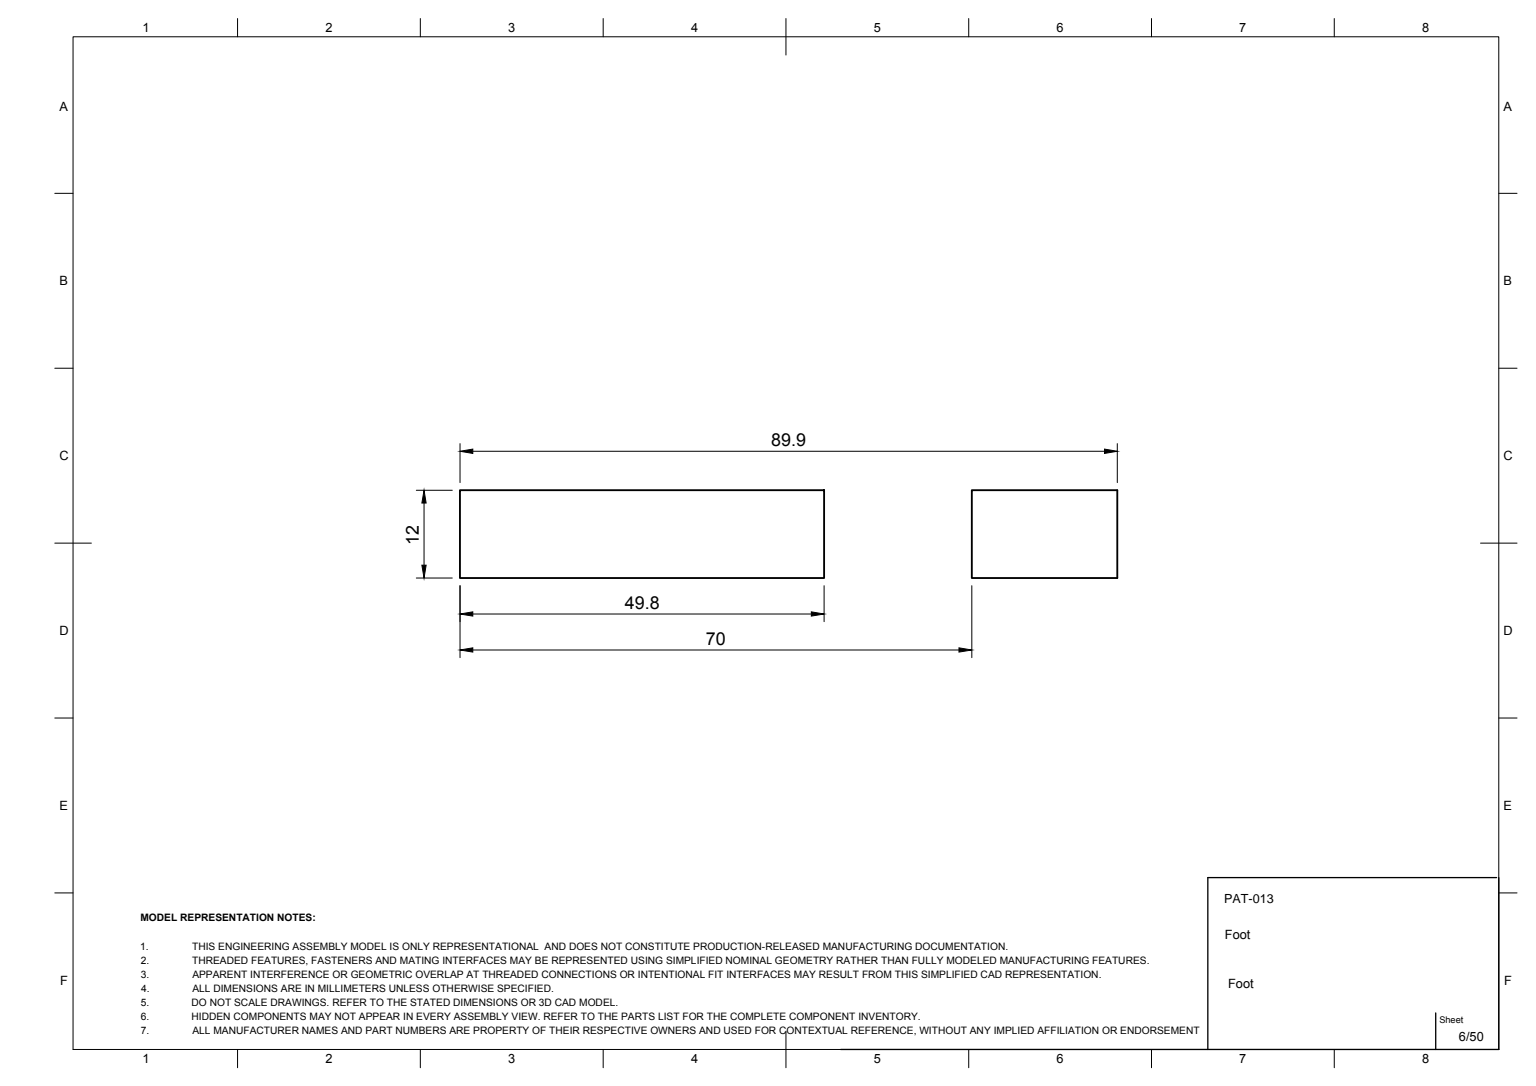
ISO-10303-21;
HEADER;
/* Generated by software containing ST-Developer
 * from STEP Tools, Inc. (www.steptools.com) 
 */

FILE_DESCRIPTION(
/* description */ ('Belt-driven linear axis on 2020 extrusion'),
/* implementation_level */ '2;1');

FILE_NAME(
/* name */ 'Foot.step',
/* time_stamp */ '2026-10-28T03:26:09-07:00',
/* author */ (''),
/* organization */ (''),
/* preprocessor_version */ 'ST-DEVELOPER v20.2',
/* originating_system */ 'Autodesk Translation Framework v15.17.0.0',
/* authorisation */ '');

FILE_SCHEMA (('AUTOMOTIVE_DESIGN { 1 0 10303 214 3 1 1 }'));
ENDSEC;

DATA;
#10=MECHANICAL_DESIGN_GEOMETRIC_PRESENTATION_REPRESENTATION('',(#611,#612),#20096);
#519=SHAPE_REPRESENTATION_RELATIONSHIP('SRR','None',#20315,#565);
#565=ADVANCED_BREP_SHAPE_REPRESENTATION('',(#667,#668),#20046);
#611=STYLED_ITEM('',(#20664),#667);
#612=STYLED_ITEM('',(#20664),#668);
#667=MANIFOLD_SOLID_BREP('Body1',#10924);
#668=MANIFOLD_SOLID_BREP('Body2',#10925);
#911=PLANE('',#11576);
#912=PLANE('',#11577);
#913=PLANE('',#11578);
#914=PLANE('',#11579);
#915=PLANE('',#11580);
#916=PLANE('',#11581);
#917=PLANE('',#11582);
#918=PLANE('',#11583);
#919=PLANE('',#11584);
#920=PLANE('',#11585);
#921=PLANE('',#11586);
#922=PLANE('',#11587);
#1292=FACE_OUTER_BOUND('',#1938,.T.);
#1293=FACE_OUTER_BOUND('',#1939,.T.);
#1294=FACE_OUTER_BOUND('',#1940,.T.);
#1295=FACE_OUTER_BOUND('',#1941,.T.);
#1296=FACE_OUTER_BOUND('',#1942,.T.);
#1297=FACE_OUTER_BOUND('',#1943,.T.);
#1298=FACE_OUTER_BOUND('',#1944,.T.);
#1299=FACE_OUTER_BOUND('',#1945,.T.);
#1300=FACE_OUTER_BOUND('',#1946,.T.);
#1301=FACE_OUTER_BOUND('',#1947,.T.);
#1302=FACE_OUTER_BOUND('',#1948,.T.);
#1303=FACE_OUTER_BOUND('',#1949,.T.);
#1938=EDGE_LOOP('',(#7397,#7398,#7399,#7400));
#1939=EDGE_LOOP('',(#7401,#7402,#7403,#7404));
#1940=EDGE_LOOP('',(#7405,#7406,#7407,#7408));
#1941=EDGE_LOOP('',(#7409,#7410,#7411,#7412));
#1942=EDGE_LOOP('',(#7413,#7414,#7415,#7416));
#1943=EDGE_LOOP('',(#7417,#7418,#7419,#7420));
#1944=EDGE_LOOP('',(#7421,#7422,#7423,#7424));
#1945=EDGE_LOOP('',(#7425,#7426,#7427,#7428));
#1946=EDGE_LOOP('',(#7429,#7430,#7431,#7432));
#1947=EDGE_LOOP('',(#7433,#7434,#7435,#7436));
#1948=EDGE_LOOP('',(#7437,#7438,#7439,#7440));
#1949=EDGE_LOOP('',(#7441,#7442,#7443,#7444));
#2697=LINE('',#16401,#3554);
#2698=LINE('',#16403,#3555);
#2699=LINE('',#16405,#3556);
#2700=LINE('',#16406,#3557);
#2701=LINE('',#16409,#3558);
#2702=LINE('',#16411,#3559);
#2703=LINE('',#16412,#3560);
#2704=LINE('',#16415,#3561);
#2705=LINE('',#16416,#3562);
#2706=LINE('',#16419,#3563);
#2707=LINE('',#16420,#3564);
#2708=LINE('',#16422,#3565);
#2709=LINE('',#16427,#3566);
#2710=LINE('',#16429,#3567);
#2711=LINE('',#16431,#3568);
#2712=LINE('',#16432,#3569);
#2713=LINE('',#16436,#3570);
#2714=LINE('',#16437,#3571);
#2715=LINE('',#16438,#3572);
#2716=LINE('',#16441,#3573);
#2717=LINE('',#16442,#3574);
#2718=LINE('',#16445,#3575);
#2719=LINE('',#16446,#3576);
#2720=LINE('',#16448,#3577);
#3554=VECTOR('',#12991,1.);
#3555=VECTOR('',#12992,1.);
#3556=VECTOR('',#12993,1.);
#3557=VECTOR('',#12994,1.);
#3558=VECTOR('',#12997,1.);
#3559=VECTOR('',#12998,1.);
#3560=VECTOR('',#12999,1.);
#3561=VECTOR('',#13002,1.);
#3562=VECTOR('',#13003,1.);
#3563=VECTOR('',#13006,1.);
#3564=VECTOR('',#13007,1.);
#3565=VECTOR('',#13010,1.);
#3566=VECTOR('',#13015,1.);
#3567=VECTOR('',#13016,1.);
#3568=VECTOR('',#13017,1.);
#3569=VECTOR('',#13018,1.);
#3570=VECTOR('',#13021,1.);
#3571=VECTOR('',#13022,1.);
#3572=VECTOR('',#13023,1.);
#3573=VECTOR('',#13026,1.);
#3574=VECTOR('',#13027,1.);
#3575=VECTOR('',#13030,1.);
#3576=VECTOR('',#13031,1.);
#3577=VECTOR('',#13034,1.);
#4940=VERTEX_POINT('',#16399);
#4941=VERTEX_POINT('',#16400);
#4942=VERTEX_POINT('',#16402);
#4943=VERTEX_POINT('',#16404);
#4944=VERTEX_POINT('',#16408);
#4945=VERTEX_POINT('',#16410);
#4946=VERTEX_POINT('',#16414);
#4947=VERTEX_POINT('',#16418);
#4948=VERTEX_POINT('',#16425);
#4949=VERTEX_POINT('',#16426);
#4950=VERTEX_POINT('',#16428);
#4951=VERTEX_POINT('',#16430);
#4952=VERTEX_POINT('',#16434);
#4953=VERTEX_POINT('',#16435);
#4954=VERTEX_POINT('',#16440);
#4955=VERTEX_POINT('',#16444);
#5913=EDGE_CURVE('',#4940,#4941,#2697,.T.);
#5914=EDGE_CURVE('',#4942,#4940,#2698,.T.);
#5915=EDGE_CURVE('',#4943,#4942,#2699,.T.);
#5916=EDGE_CURVE('',#4941,#4943,#2700,.T.);
#5917=EDGE_CURVE('',#4942,#4944,#2701,.T.);
#5918=EDGE_CURVE('',#4944,#4945,#2702,.T.);
#5919=EDGE_CURVE('',#4945,#4943,#2703,.T.);
#5920=EDGE_CURVE('',#4940,#4946,#2704,.T.);
#5921=EDGE_CURVE('',#4946,#4944,#2705,.T.);
#5922=EDGE_CURVE('',#4947,#4946,#2706,.T.);
#5923=EDGE_CURVE('',#4945,#4947,#2707,.T.);
#5924=EDGE_CURVE('',#4947,#4941,#2708,.T.);
#5925=EDGE_CURVE('',#4948,#4949,#2709,.T.);
#5926=EDGE_CURVE('',#4949,#4950,#2710,.T.);
#5927=EDGE_CURVE('',#4951,#4950,#2711,.T.);
#5928=EDGE_CURVE('',#4948,#4951,#2712,.T.);
#5929=EDGE_CURVE('',#4952,#4953,#2713,.T.);
#5930=EDGE_CURVE('',#4953,#4948,#2714,.T.);
#5931=EDGE_CURVE('',#4952,#4951,#2715,.T.);
#5932=EDGE_CURVE('',#4954,#4952,#2716,.T.);
#5933=EDGE_CURVE('',#4950,#4954,#2717,.T.);
#5934=EDGE_CURVE('',#4955,#4954,#2718,.T.);
#5935=EDGE_CURVE('',#4949,#4955,#2719,.T.);
#5936=EDGE_CURVE('',#4953,#4955,#2720,.T.);
#7397=ORIENTED_EDGE('',*,*,#5913,.F.);
#7398=ORIENTED_EDGE('',*,*,#5914,.F.);
#7399=ORIENTED_EDGE('',*,*,#5915,.F.);
#7400=ORIENTED_EDGE('',*,*,#5916,.F.);
#7401=ORIENTED_EDGE('',*,*,#5915,.T.);
#7402=ORIENTED_EDGE('',*,*,#5917,.T.);
#7403=ORIENTED_EDGE('',*,*,#5918,.T.);
#7404=ORIENTED_EDGE('',*,*,#5919,.T.);
#7405=ORIENTED_EDGE('',*,*,#5914,.T.);
#7406=ORIENTED_EDGE('',*,*,#5920,.T.);
#7407=ORIENTED_EDGE('',*,*,#5921,.T.);
#7408=ORIENTED_EDGE('',*,*,#5917,.F.);
#7409=ORIENTED_EDGE('',*,*,#5921,.F.);
#7410=ORIENTED_EDGE('',*,*,#5922,.F.);
#7411=ORIENTED_EDGE('',*,*,#5923,.F.);
#7412=ORIENTED_EDGE('',*,*,#5918,.F.);
#7413=ORIENTED_EDGE('',*,*,#5913,.T.);
#7414=ORIENTED_EDGE('',*,*,#5924,.F.);
#7415=ORIENTED_EDGE('',*,*,#5922,.T.);
#7416=ORIENTED_EDGE('',*,*,#5920,.F.);
#7417=ORIENTED_EDGE('',*,*,#5916,.T.);
#7418=ORIENTED_EDGE('',*,*,#5919,.F.);
#7419=ORIENTED_EDGE('',*,*,#5923,.T.);
#7420=ORIENTED_EDGE('',*,*,#5924,.T.);
#7421=ORIENTED_EDGE('',*,*,#5925,.T.);
#7422=ORIENTED_EDGE('',*,*,#5926,.T.);
#7423=ORIENTED_EDGE('',*,*,#5927,.F.);
#7424=ORIENTED_EDGE('',*,*,#5928,.F.);
#7425=ORIENTED_EDGE('',*,*,#5929,.T.);
#7426=ORIENTED_EDGE('',*,*,#5930,.T.);
#7427=ORIENTED_EDGE('',*,*,#5928,.T.);
#7428=ORIENTED_EDGE('',*,*,#5931,.F.);
#7429=ORIENTED_EDGE('',*,*,#5932,.T.);
#7430=ORIENTED_EDGE('',*,*,#5931,.T.);
#7431=ORIENTED_EDGE('',*,*,#5927,.T.);
#7432=ORIENTED_EDGE('',*,*,#5933,.T.);
#7433=ORIENTED_EDGE('',*,*,#5934,.T.);
#7434=ORIENTED_EDGE('',*,*,#5933,.F.);
#7435=ORIENTED_EDGE('',*,*,#5926,.F.);
#7436=ORIENTED_EDGE('',*,*,#5935,.T.);
#7437=ORIENTED_EDGE('',*,*,#5936,.T.);
#7438=ORIENTED_EDGE('',*,*,#5935,.F.);
#7439=ORIENTED_EDGE('',*,*,#5925,.F.);
#7440=ORIENTED_EDGE('',*,*,#5930,.F.);
#7441=ORIENTED_EDGE('',*,*,#5929,.F.);
#7442=ORIENTED_EDGE('',*,*,#5932,.F.);
#7443=ORIENTED_EDGE('',*,*,#5934,.F.);
#7444=ORIENTED_EDGE('',*,*,#5936,.F.);
#10343=ADVANCED_FACE('',(#1292),#911,.F.);
#10344=ADVANCED_FACE('',(#1293),#912,.T.);
#10345=ADVANCED_FACE('',(#1294),#913,.T.);
#10346=ADVANCED_FACE('',(#1295),#914,.F.);
#10347=ADVANCED_FACE('',(#1296),#915,.F.);
#10348=ADVANCED_FACE('',(#1297),#916,.T.);
#10349=ADVANCED_FACE('',(#1298),#917,.T.);
#10350=ADVANCED_FACE('',(#1299),#918,.T.);
#10351=ADVANCED_FACE('',(#1300),#919,.T.);
#10352=ADVANCED_FACE('',(#1301),#920,.T.);
#10353=ADVANCED_FACE('',(#1302),#921,.F.);
#10354=ADVANCED_FACE('',(#1303),#922,.F.);
#10924=CLOSED_SHELL('',(#10343,#10344,#10345,#10346,#10347,#10348));
#10925=CLOSED_SHELL('',(#10349,#10350,#10351,#10352,#10353,#10354));
#11575=AXIS2_PLACEMENT_3D('',#16397,#12987,#12988);
#11576=AXIS2_PLACEMENT_3D('',#16398,#12989,#12990);
#11577=AXIS2_PLACEMENT_3D('',#16407,#12995,#12996);
#11578=AXIS2_PLACEMENT_3D('',#16413,#13000,#13001);
#11579=AXIS2_PLACEMENT_3D('',#16417,#13004,#13005);
#11580=AXIS2_PLACEMENT_3D('',#16421,#13008,#13009);
#11581=AXIS2_PLACEMENT_3D('',#16423,#13011,#13012);
#11582=AXIS2_PLACEMENT_3D('',#16424,#13013,#13014);
#11583=AXIS2_PLACEMENT_3D('',#16433,#13019,#13020);
#11584=AXIS2_PLACEMENT_3D('',#16439,#13024,#13025);
#11585=AXIS2_PLACEMENT_3D('',#16443,#13028,#13029);
#11586=AXIS2_PLACEMENT_3D('',#16447,#13032,#13033);
#11587=AXIS2_PLACEMENT_3D('',#16449,#13035,#13036);
#12987=DIRECTION('axis',(0.,0.,1.));
#12988=DIRECTION('refdir',(1.,0.,0.));
#12989=DIRECTION('center_axis',(0.,-1.,0.));
#12990=DIRECTION('ref_axis',(1.,0.,0.));
#12991=DIRECTION('',(1.,0.,0.));
#12992=DIRECTION('',(0.,0.,-1.));
#12993=DIRECTION('',(-1.,0.,0.));
#12994=DIRECTION('',(0.,0.,1.));
#12995=DIRECTION('center_axis',(0.,0.,1.));
#12996=DIRECTION('ref_axis',(1.,0.,0.));
#12997=DIRECTION('',(0.,-1.,0.));
#12998=DIRECTION('',(1.,0.,0.));
#12999=DIRECTION('',(0.,1.,0.));
#13000=DIRECTION('center_axis',(-1.,0.,0.));
#13001=DIRECTION('ref_axis',(0.,-1.,0.));
#13002=DIRECTION('',(0.,-1.,0.));
#13003=DIRECTION('',(0.,0.,1.));
#13004=DIRECTION('center_axis',(0.,1.,0.));
#13005=DIRECTION('ref_axis',(-1.,0.,0.));
#13006=DIRECTION('',(-1.,0.,0.));
#13007=DIRECTION('',(0.,0.,-1.));
#13008=DIRECTION('center_axis',(0.,0.,1.));
#13009=DIRECTION('ref_axis',(1.,0.,0.));
#13010=DIRECTION('',(0.,1.,0.));
#13011=DIRECTION('center_axis',(1.,0.,0.));
#13012=DIRECTION('ref_axis',(0.,1.,0.));
#13013=DIRECTION('center_axis',(0.,-1.,0.));
#13014=DIRECTION('ref_axis',(1.,0.,0.));
#13015=DIRECTION('',(1.,0.,0.));
#13016=DIRECTION('',(0.,0.,1.));
#13017=DIRECTION('',(1.,0.,0.));
#13018=DIRECTION('',(0.,0.,1.));
#13019=DIRECTION('center_axis',(-1.,0.,0.));
#13020=DIRECTION('ref_axis',(0.,-1.,0.));
#13021=DIRECTION('',(0.,0.,-1.));
#13022=DIRECTION('',(0.,-1.,0.));
#13023=DIRECTION('',(0.,-1.,0.));
#13024=DIRECTION('center_axis',(0.,0.,1.));
#13025=DIRECTION('ref_axis',(1.,0.,0.));
#13026=DIRECTION('',(-1.,0.,0.));
#13027=DIRECTION('',(0.,1.,0.));
#13028=DIRECTION('center_axis',(1.,0.,0.));
#13029=DIRECTION('ref_axis',(0.,1.,0.));
#13030=DIRECTION('',(0.,0.,1.));
#13031=DIRECTION('',(0.,1.,0.));
#13032=DIRECTION('center_axis',(0.,0.,1.));
#13033=DIRECTION('ref_axis',(1.,0.,0.));
#13034=DIRECTION('',(1.,0.,0.));
#13035=DIRECTION('center_axis',(0.,-1.,0.));
#13036=DIRECTION('ref_axis',(1.,0.,0.));
#16397=CARTESIAN_POINT('',(0.,0.,0.));
#16398=CARTESIAN_POINT('Origin',(-4.1,2.49,-2.5));
#16399=CARTESIAN_POINT('',(-4.,2.49,-2.4));
#16400=CARTESIAN_POINT('',(-3.,2.49,-2.4));
#16401=CARTESIAN_POINT('',(-3.8,2.49,-2.4));
#16402=CARTESIAN_POINT('',(-4.,2.49,-1.2));
#16403=CARTESIAN_POINT('',(-4.,2.49,-2.45));
#16404=CARTESIAN_POINT('',(-3.,2.49,-1.2));
#16405=CARTESIAN_POINT('',(-3.8,2.49,-1.2));
#16406=CARTESIAN_POINT('',(-3.,2.49,-2.45));
#16407=CARTESIAN_POINT('Origin',(-3.5,-1.,-1.2));
#16408=CARTESIAN_POINT('',(-4.,-2.49,-1.2));
#16409=CARTESIAN_POINT('',(-4.,4.5,-1.2));
#16410=CARTESIAN_POINT('',(-3.,-2.49,-1.2));
#16411=CARTESIAN_POINT('',(16.3,-2.49,-1.2));
#16412=CARTESIAN_POINT('',(-3.,-6.5,-1.2));
#16413=CARTESIAN_POINT('Origin',(-4.,4.5,-2.4));
#16414=CARTESIAN_POINT('',(-4.,-2.49,-2.4));
#16415=CARTESIAN_POINT('',(-4.,4.5,-2.4));
#16416=CARTESIAN_POINT('',(-4.,-2.49,-2.45));
#16417=CARTESIAN_POINT('Origin',(36.1,-2.49,-2.5));
#16418=CARTESIAN_POINT('',(-3.,-2.49,-2.4));
#16419=CARTESIAN_POINT('',(16.3,-2.49,-2.4));
#16420=CARTESIAN_POINT('',(-3.,-2.49,-2.45));
#16421=CARTESIAN_POINT('Origin',(-3.5,-1.,-2.4));
#16422=CARTESIAN_POINT('',(-3.,-6.5,-2.4));
#16423=CARTESIAN_POINT('Origin',(-3.,-6.5,-2.4));
#16424=CARTESIAN_POINT('Origin',(-4.,-6.5,-2.4));
#16425=CARTESIAN_POINT('',(-4.,-6.5,-2.4));
#16426=CARTESIAN_POINT('',(-3.,-6.5,-2.4));
#16427=CARTESIAN_POINT('',(-4.,-6.5,-2.4));
#16428=CARTESIAN_POINT('',(-3.,-6.5,-1.2));
#16429=CARTESIAN_POINT('',(-3.,-6.5,-2.4));
#16430=CARTESIAN_POINT('',(-4.,-6.5,-1.2));
#16431=CARTESIAN_POINT('',(-4.,-6.5,-1.2));
#16432=CARTESIAN_POINT('',(-4.,-6.5,-2.4));
#16433=CARTESIAN_POINT('Origin',(-4.,4.5,-2.4));
#16434=CARTESIAN_POINT('',(-4.,-4.51,-1.2));
#16435=CARTESIAN_POINT('',(-4.,-4.51,-2.4));
#16436=CARTESIAN_POINT('',(-4.,-4.51,-2.45));
#16437=CARTESIAN_POINT('',(-4.,4.5,-2.4));
#16438=CARTESIAN_POINT('',(-4.,4.5,-1.2));
#16439=CARTESIAN_POINT('Origin',(-3.5,-1.,-1.2));
#16440=CARTESIAN_POINT('',(-3.,-4.51,-1.2));
#16441=CARTESIAN_POINT('',(-3.8,-4.51,-1.2));
#16442=CARTESIAN_POINT('',(-3.,-6.5,-1.2));
#16443=CARTESIAN_POINT('Origin',(-3.,-6.5,-2.4));
#16444=CARTESIAN_POINT('',(-3.,-4.51,-2.4));
#16445=CARTESIAN_POINT('',(-3.,-4.51,-2.45));
#16446=CARTESIAN_POINT('',(-3.,-6.5,-2.4));
#16447=CARTESIAN_POINT('Origin',(-3.5,-1.,-2.4));
#16448=CARTESIAN_POINT('',(-3.8,-4.51,-2.4));
#16449=CARTESIAN_POINT('Origin',(-4.1,-4.51,-2.5));
#19992=UNCERTAINTY_MEASURE_WITH_UNIT(LENGTH_MEASURE(0.001),#20097,
'DISTANCE_ACCURACY_VALUE',
'Maximum model space distance between geometric entities at asserted c
onnectivities');
#20042=UNCERTAINTY_MEASURE_WITH_UNIT(LENGTH_MEASURE(0.001),#20097,
'DISTANCE_ACCURACY_VALUE',
'Maximum model space distance between geometric entities at asserted c
onnectivities');
#20046=(
GEOMETRIC_REPRESENTATION_CONTEXT(3)
GLOBAL_UNCERTAINTY_ASSIGNED_CONTEXT((#19992))
GLOBAL_UNIT_ASSIGNED_CONTEXT((#20097,#20099,#20100))
REPRESENTATION_CONTEXT('','3D')
);
#20096=(
GEOMETRIC_REPRESENTATION_CONTEXT(3)
GLOBAL_UNCERTAINTY_ASSIGNED_CONTEXT((#20042))
GLOBAL_UNIT_ASSIGNED_CONTEXT((#20097,#20099,#20100))
REPRESENTATION_CONTEXT('','3D')
);
#20097=(
LENGTH_UNIT()
NAMED_UNIT(*)
SI_UNIT(.CENTI.,.METRE.)
);
#20099=(
NAMED_UNIT(*)
PLANE_ANGLE_UNIT()
SI_UNIT($,.RADIAN.)
);
#20100=(
NAMED_UNIT(*)
SI_UNIT($,.STERADIAN.)
SOLID_ANGLE_UNIT()
);
#20104=SHAPE_DEFINITION_REPRESENTATION(#20157,#20315);
#20157=PRODUCT_DEFINITION_SHAPE('',$,#20369);
#20315=SHAPE_REPRESENTATION('',(#11575),#20046);
#20365=PRODUCT_DEFINITION_CONTEXT('part definition',#20526,'design');
#20369=PRODUCT_DEFINITION('Foot','Foot',#20422,#20365);
#20422=PRODUCT_DEFINITION_FORMATION('',$,#20531);
#20526=APPLICATION_CONTEXT(
'Core Data for Automotive Mechanical Design Process');
#20527=PRODUCT_CONTEXT('part definition',#20526,'mechanical');
#20531=PRODUCT('Foot','Foot','Foot',(#20527));
#20658=COLOUR_RGB('Off White',0.89,0.88,0.83);
#20659=FILL_AREA_STYLE_COLOUR('',#20658);
#20660=FILL_AREA_STYLE('',(#20659));
#20661=SURFACE_STYLE_FILL_AREA(#20660);
#20662=SURFACE_SIDE_STYLE('',(#20661));
#20663=SURFACE_STYLE_USAGE(.BOTH.,#20662);
#20664=PRESENTATION_STYLE_ASSIGNMENT((#20663));
ENDSEC;
END-ISO-10303-21;
